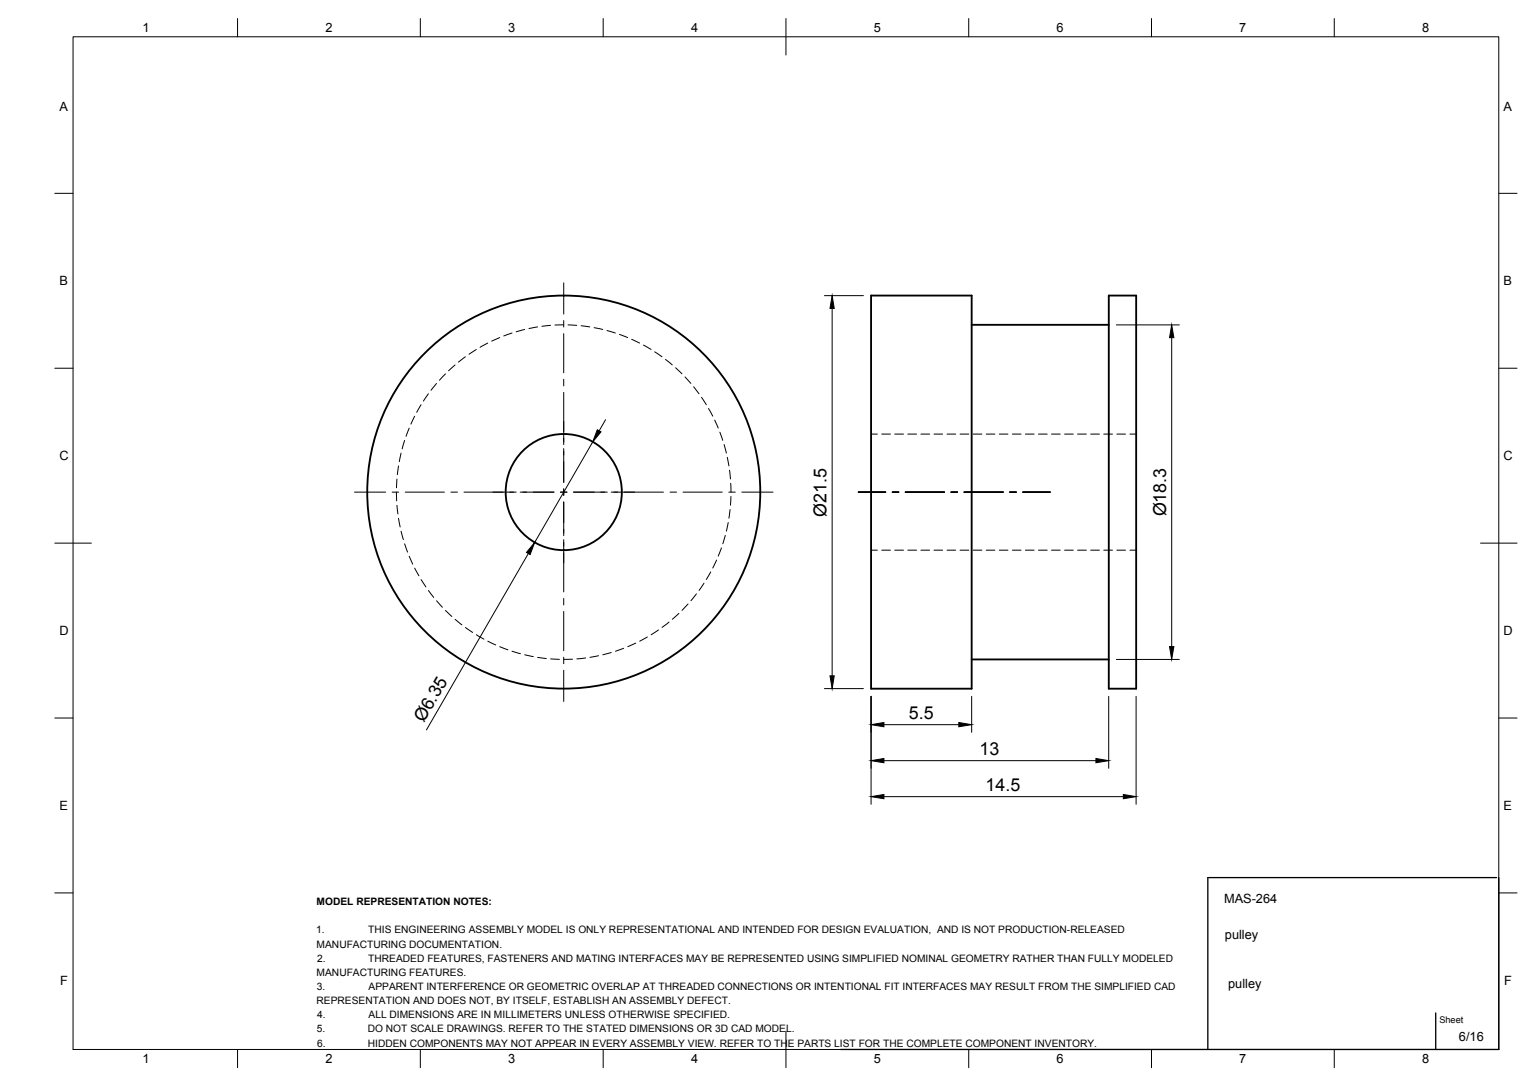
ISO-10303-21;
HEADER;
/* Generated by software containing ST-Developer
 * from STEP Tools, Inc. (www.steptools.com) 
 */

FILE_DESCRIPTION(
/* description */ (''),
/* implementation_level */ '2;1');

FILE_NAME(
/* name */ 'Pulley.step',
/* time_stamp */ '2026-10-12T15:37:13-07:00',
/* author */ (''),
/* organization */ (''),
/* preprocessor_version */ 'ST-DEVELOPER v20.2',
/* originating_system */ 'Autodesk Translation Framework v15.15.0.0',
/* authorisation */ '');

FILE_SCHEMA (('AUTOMOTIVE_DESIGN { 1 0 10303 214 3 1 1 }'));
ENDSEC;

DATA;
#10=MECHANICAL_DESIGN_GEOMETRIC_PRESENTATION_REPRESENTATION('',(#351),#36460);
#112=SHAPE_REPRESENTATION_RELATIONSHIP('SRR','None',#36524,#125);
#125=ADVANCED_BREP_SHAPE_REPRESENTATION('',(#383),#36453);
#178=FACE_BOUND('',#2146,.T.);
#179=FACE_BOUND('',#2149,.T.);
#180=FACE_BOUND('',#2151,.T.);
#181=FACE_BOUND('',#2155,.T.);
#351=STYLED_ITEM('',(#36598),#383);
#383=MANIFOLD_SOLID_BREP('Body1',#11287);
#630=PLANE('',#12119);
#631=PLANE('',#12125);
#632=PLANE('',#12127);
#633=PLANE('',#12132);
#1485=FACE_OUTER_BOUND('',#2145,.T.);
#1486=FACE_OUTER_BOUND('',#2147,.T.);
#1487=FACE_OUTER_BOUND('',#2148,.T.);
#1488=FACE_OUTER_BOUND('',#2150,.T.);
#1489=FACE_OUTER_BOUND('',#2152,.T.);
#1490=FACE_OUTER_BOUND('',#2153,.T.);
#1491=FACE_OUTER_BOUND('',#2154,.T.);
#1492=FACE_OUTER_BOUND('',#2156,.T.);
#2145=EDGE_LOOP('',(#9614));
#2146=EDGE_LOOP('',(#9615));
#2147=EDGE_LOOP('',(#9616,#9617,#9618,#9619));
#2148=EDGE_LOOP('',(#9620));
#2149=EDGE_LOOP('',(#9621));
#2150=EDGE_LOOP('',(#9622));
#2151=EDGE_LOOP('',(#9623));
#2152=EDGE_LOOP('',(#9624,#9625,#9626,#9627));
#2153=EDGE_LOOP('',(#9628,#9629,#9630,#9631));
#2154=EDGE_LOOP('',(#9632));
#2155=EDGE_LOOP('',(#9633));
#2156=EDGE_LOOP('',(#9634,#9635,#9636,#9637));
#3082=LINE('',#35461,#4028);
#3083=LINE('',#35471,#4029);
#3084=LINE('',#35474,#4030);
#3085=LINE('',#35479,#4031);
#4028=VECTOR('',#14503,9.15);
#4029=VECTOR('',#14516,10.75);
#4030=VECTOR('',#14521,10.75);
#4031=VECTOR('',#14528,3.17500000000003);
#4453=CIRCLE('',#12120,10.75);
#4454=CIRCLE('',#12121,3.17500000000003);
#4455=CIRCLE('',#12123,9.15);
#4456=CIRCLE('',#12124,9.15);
#4457=CIRCLE('',#12126,10.75);
#4458=CIRCLE('',#12128,10.75);
#4459=CIRCLE('',#12130,10.75);
#4460=CIRCLE('',#12133,3.17500000000003);
#5387=VERTEX_POINT('',#35453);
#5388=VERTEX_POINT('',#35455);
#5389=VERTEX_POINT('',#35458);
#5390=VERTEX_POINT('',#35460);
#5391=VERTEX_POINT('',#35464);
#5392=VERTEX_POINT('',#35467);
#5393=VERTEX_POINT('',#35470);
#5394=VERTEX_POINT('',#35476);
#6838=EDGE_CURVE('',#5387,#5387,#4453,.T.);
#6839=EDGE_CURVE('',#5388,#5388,#4454,.T.);
#6840=EDGE_CURVE('',#5389,#5389,#4455,.T.);
#6841=EDGE_CURVE('',#5389,#5390,#3082,.T.);
#6842=EDGE_CURVE('',#5390,#5390,#4456,.F.);
#6843=EDGE_CURVE('',#5391,#5391,#4457,.T.);
#6844=EDGE_CURVE('',#5392,#5392,#4458,.T.);
#6845=EDGE_CURVE('',#5391,#5393,#3083,.T.);
#6846=EDGE_CURVE('',#5393,#5393,#4459,.T.);
#6847=EDGE_CURVE('',#5387,#5392,#3084,.T.);
#6848=EDGE_CURVE('',#5394,#5394,#4460,.T.);
#6849=EDGE_CURVE('',#5394,#5388,#3085,.T.);
#9614=ORIENTED_EDGE('',*,*,#6838,.T.);
#9615=ORIENTED_EDGE('',*,*,#6839,.T.);
#9616=ORIENTED_EDGE('',*,*,#6840,.F.);
#9617=ORIENTED_EDGE('',*,*,#6841,.T.);
#9618=ORIENTED_EDGE('',*,*,#6842,.F.);
#9619=ORIENTED_EDGE('',*,*,#6841,.F.);
#9620=ORIENTED_EDGE('',*,*,#6843,.T.);
#9621=ORIENTED_EDGE('',*,*,#6842,.T.);
#9622=ORIENTED_EDGE('',*,*,#6844,.F.);
#9623=ORIENTED_EDGE('',*,*,#6840,.T.);
#9624=ORIENTED_EDGE('',*,*,#6843,.F.);
#9625=ORIENTED_EDGE('',*,*,#6845,.T.);
#9626=ORIENTED_EDGE('',*,*,#6846,.T.);
#9627=ORIENTED_EDGE('',*,*,#6845,.F.);
#9628=ORIENTED_EDGE('',*,*,#6838,.F.);
#9629=ORIENTED_EDGE('',*,*,#6847,.T.);
#9630=ORIENTED_EDGE('',*,*,#6844,.T.);
#9631=ORIENTED_EDGE('',*,*,#6847,.F.);
#9632=ORIENTED_EDGE('',*,*,#6846,.F.);
#9633=ORIENTED_EDGE('',*,*,#6848,.F.);
#9634=ORIENTED_EDGE('',*,*,#6848,.T.);
#9635=ORIENTED_EDGE('',*,*,#6849,.T.);
#9636=ORIENTED_EDGE('',*,*,#6839,.F.);
#9637=ORIENTED_EDGE('',*,*,#6849,.F.);
#10579=CYLINDRICAL_SURFACE('',#12122,9.15);
#10580=CYLINDRICAL_SURFACE('',#12129,10.75);
#10581=CYLINDRICAL_SURFACE('',#12131,10.75);
#10582=CYLINDRICAL_SURFACE('',#12134,3.17500000000003);
#11106=ADVANCED_FACE('',(#1485,#178),#630,.T.);
#11107=ADVANCED_FACE('',(#1486),#10579,.T.);
#11108=ADVANCED_FACE('',(#1487,#179),#631,.T.);
#11109=ADVANCED_FACE('',(#1488,#180),#632,.F.);
#11110=ADVANCED_FACE('',(#1489),#10580,.T.);
#11111=ADVANCED_FACE('',(#1490),#10581,.T.);
#11112=ADVANCED_FACE('',(#1491,#181),#633,.F.);
#11113=ADVANCED_FACE('',(#1492),#10582,.F.);
#11287=CLOSED_SHELL('',(#11106,#11107,#11108,#11109,#11110,#11111,#11112,
#11113));
#12118=AXIS2_PLACEMENT_3D('',#35451,#14491,#14492);
#12119=AXIS2_PLACEMENT_3D('',#35452,#14493,#14494);
#12120=AXIS2_PLACEMENT_3D('',#35454,#14495,#14496);
#12121=AXIS2_PLACEMENT_3D('',#35456,#14497,#14498);
#12122=AXIS2_PLACEMENT_3D('',#35457,#14499,#14500);
#12123=AXIS2_PLACEMENT_3D('',#35459,#14501,#14502);
#12124=AXIS2_PLACEMENT_3D('',#35462,#14504,#14505);
#12125=AXIS2_PLACEMENT_3D('',#35463,#14506,#14507);
#12126=AXIS2_PLACEMENT_3D('',#35465,#14508,#14509);
#12127=AXIS2_PLACEMENT_3D('',#35466,#14510,#14511);
#12128=AXIS2_PLACEMENT_3D('',#35468,#14512,#14513);
#12129=AXIS2_PLACEMENT_3D('',#35469,#14514,#14515);
#12130=AXIS2_PLACEMENT_3D('',#35472,#14517,#14518);
#12131=AXIS2_PLACEMENT_3D('',#35473,#14519,#14520);
#12132=AXIS2_PLACEMENT_3D('',#35475,#14522,#14523);
#12133=AXIS2_PLACEMENT_3D('',#35477,#14524,#14525);
#12134=AXIS2_PLACEMENT_3D('',#35478,#14526,#14527);
#14491=DIRECTION('axis',(0.,0.,1.));
#14492=DIRECTION('refdir',(1.,0.,0.));
#14493=DIRECTION('center_axis',(2.24770354660149E-47,-8.64291075969854E-33,
1.));
#14494=DIRECTION('ref_axis',(1.,1.12331423616832E-95,-2.24770354660149E-47));
#14495=DIRECTION('center_axis',(-1.97812547909132E-47,-3.45804190325652E-32,
1.));
#14496=DIRECTION('ref_axis',(1.,-3.6491105917259E-95,1.97812547909132E-47));
#14497=DIRECTION('center_axis',(-2.24770354660149E-47,8.64291075969854E-33,
-1.));
#14498=DIRECTION('ref_axis',(1.,1.94267011675346E-79,-2.24770354660149E-47));
#14499=DIRECTION('center_axis',(0.,0.,1.));
#14500=DIRECTION('ref_axis',(1.,0.,0.));
#14501=DIRECTION('center_axis',(-9.86076131526267E-32,5.23079214264925E-32,
1.));
#14502=DIRECTION('ref_axis',(1.,-4.21761455916246E-79,9.86076131526267E-32));
#14503=DIRECTION('',(0.,0.,-1.));
#14504=DIRECTION('center_axis',(-1.97812547909132E-47,-3.45804190325652E-32,
1.));
#14505=DIRECTION('ref_axis',(1.,-6.84044079659716E-79,1.97812547909132E-47));
#14506=DIRECTION('center_axis',(-1.97812547909132E-47,-3.45804190325652E-32,
1.));
#14507=DIRECTION('ref_axis',(1.,-3.6491105917259E-95,1.97812547909132E-47));
#14508=DIRECTION('center_axis',(-1.97812547909132E-47,-3.45804190325652E-32,
1.));
#14509=DIRECTION('ref_axis',(1.,-6.84044079659716E-79,1.97812547909132E-47));
#14510=DIRECTION('center_axis',(-1.97812547909132E-47,-3.45804190325652E-32,
1.));
#14511=DIRECTION('ref_axis',(1.,-3.6491105917259E-95,1.97812547909132E-47));
#14512=DIRECTION('center_axis',(-1.97812547909132E-47,-3.45804190325652E-32,
1.));
#14513=DIRECTION('ref_axis',(1.,-3.6491105917259E-95,1.97812547909132E-47));
#14514=DIRECTION('center_axis',(0.,0.,1.));
#14515=DIRECTION('ref_axis',(1.,0.,0.));
#14516=DIRECTION('',(0.,0.,-1.));
#14517=DIRECTION('center_axis',(-1.97812547909132E-47,-3.45804190325652E-32,
1.));
#14518=DIRECTION('ref_axis',(1.,-6.84044079659716E-79,1.97812547909132E-47));
#14519=DIRECTION('center_axis',(0.,0.,1.));
#14520=DIRECTION('ref_axis',(1.,0.,0.));
#14521=DIRECTION('',(0.,0.,-1.));
#14522=DIRECTION('center_axis',(-1.97812547909132E-47,-3.45804190325652E-32,
1.));
#14523=DIRECTION('ref_axis',(1.,-3.6491105917259E-95,1.97812547909132E-47));
#14524=DIRECTION('center_axis',(1.97812547909132E-47,3.45804190325652E-32,
-1.));
#14525=DIRECTION('ref_axis',(1.,-6.84044079659716E-79,1.97812547909132E-47));
#14526=DIRECTION('center_axis',(0.,0.,1.));
#14527=DIRECTION('ref_axis',(1.,0.,0.));
#14528=DIRECTION('',(0.,0.,1.));
#35451=CARTESIAN_POINT('',(0.,0.,0.));
#35452=CARTESIAN_POINT('Origin',(-10.,520.056498641762,4.99200000000021));
#35453=CARTESIAN_POINT('',(-20.75,520.056498641762,4.99200000000021));
#35454=CARTESIAN_POINT('Origin',(-10.,520.056498641762,4.99200000000021));
#35455=CARTESIAN_POINT('',(-13.175,520.056498641762,4.99200000000021));
#35456=CARTESIAN_POINT('Origin',(-9.99999999999998,520.056498641762,4.99200000000021));
#35457=CARTESIAN_POINT('Origin',(-9.99999999999996,520.056498641762,-3.50799999999979));
#35458=CARTESIAN_POINT('',(-19.15,520.056498641762,3.49200000000021));
#35459=CARTESIAN_POINT('Origin',(-9.99999999999996,520.056498641762,3.49200000000021));
#35460=CARTESIAN_POINT('',(-19.15,520.056498641762,-4.00799999999979));
#35461=CARTESIAN_POINT('',(-19.15,520.056498641762,-3.50799999999979));
#35462=CARTESIAN_POINT('Origin',(-9.99999999999996,520.056498641762,-4.00799999999979));
#35463=CARTESIAN_POINT('Origin',(-10.,520.056498641762,-4.00799999999979));
#35464=CARTESIAN_POINT('',(-20.75,520.056498641762,-4.00799999999979));
#35465=CARTESIAN_POINT('Origin',(-10.,520.056498641762,-4.00799999999979));
#35466=CARTESIAN_POINT('Origin',(-10.,520.056498641762,3.49200000000021));
#35467=CARTESIAN_POINT('',(-20.75,520.056498641762,3.49200000000021));
#35468=CARTESIAN_POINT('Origin',(-10.,520.056498641762,3.49200000000021));
#35469=CARTESIAN_POINT('Origin',(-10.,520.056498641762,-3.50799999999979));
#35470=CARTESIAN_POINT('',(-20.75,520.056498641762,-9.50799999999979));
#35471=CARTESIAN_POINT('',(-20.75,520.056498641762,-3.50799999999979));
#35472=CARTESIAN_POINT('Origin',(-10.,520.056498641762,-9.50799999999979));
#35473=CARTESIAN_POINT('Origin',(-10.,520.056498641762,3.49200000000021));
#35474=CARTESIAN_POINT('',(-20.75,520.056498641762,3.49200000000021));
#35475=CARTESIAN_POINT('Origin',(-10.,520.056498641762,-9.50799999999979));
#35476=CARTESIAN_POINT('',(-13.175,520.056498641762,-9.50799999999979));
#35477=CARTESIAN_POINT('Origin',(-9.99999999999998,520.056498641762,-9.50799999999979));
#35478=CARTESIAN_POINT('Origin',(-9.99999999999998,520.056498641762,-3.50799999999979));
#35479=CARTESIAN_POINT('',(-13.175,520.056498641762,-3.50799999999979));
#36437=UNCERTAINTY_MEASURE_WITH_UNIT(LENGTH_MEASURE(0.01),#36461,
'DISTANCE_ACCURACY_VALUE',
'Maximum model space distance between geometric entities at asserted c
onnectivities');
#36444=UNCERTAINTY_MEASURE_WITH_UNIT(LENGTH_MEASURE(0.01),#36461,
'DISTANCE_ACCURACY_VALUE',
'Maximum model space distance between geometric entities at asserted c
onnectivities');
#36453=(
GEOMETRIC_REPRESENTATION_CONTEXT(3)
GLOBAL_UNCERTAINTY_ASSIGNED_CONTEXT((#36437))
GLOBAL_UNIT_ASSIGNED_CONTEXT((#36461,#36463,#36464))
REPRESENTATION_CONTEXT('','3D')
);
#36460=(
GEOMETRIC_REPRESENTATION_CONTEXT(3)
GLOBAL_UNCERTAINTY_ASSIGNED_CONTEXT((#36444))
GLOBAL_UNIT_ASSIGNED_CONTEXT((#36461,#36463,#36464))
REPRESENTATION_CONTEXT('','3D')
);
#36461=(
LENGTH_UNIT()
NAMED_UNIT(*)
SI_UNIT(.MILLI.,.METRE.)
);
#36463=(
NAMED_UNIT(*)
PLANE_ANGLE_UNIT()
SI_UNIT($,.RADIAN.)
);
#36464=(
NAMED_UNIT(*)
SI_UNIT($,.STERADIAN.)
SOLID_ANGLE_UNIT()
);
#36473=SHAPE_DEFINITION_REPRESENTATION(#36493,#36524);
#36493=PRODUCT_DEFINITION_SHAPE('',$,#36540);
#36524=SHAPE_REPRESENTATION('',(#12118),#36453);
#36531=PRODUCT_DEFINITION_CONTEXT('part definition',#36578,'design');
#36540=PRODUCT_DEFINITION('pulley','Pulley',#36555,#36531);
#36555=PRODUCT_DEFINITION_FORMATION('',$,#36588);
#36578=APPLICATION_CONTEXT(
'Core Data for Automotive Mechanical Design Process');
#36579=PRODUCT_CONTEXT('part definition',#36578,'mechanical');
#36588=PRODUCT('pulley','Pulley',$,(#36579));
#36598=PRESENTATION_STYLE_ASSIGNMENT((#36603));
#36603=SURFACE_STYLE_USAGE(.BOTH.,#36608);
#36608=SURFACE_SIDE_STYLE('',(#36613));
#36613=SURFACE_STYLE_FILL_AREA(#36618);
#36618=FILL_AREA_STYLE('Opaque(245,245,246)',(#36623));
#36623=FILL_AREA_STYLE_COLOUR('Opaque(245,245,246)',#36628);
#36628=COLOUR_RGB('Opaque(245,245,246)', 0.40784314, 0.44705882, 0.49803922);
ENDSEC;
END-ISO-10303-21;
